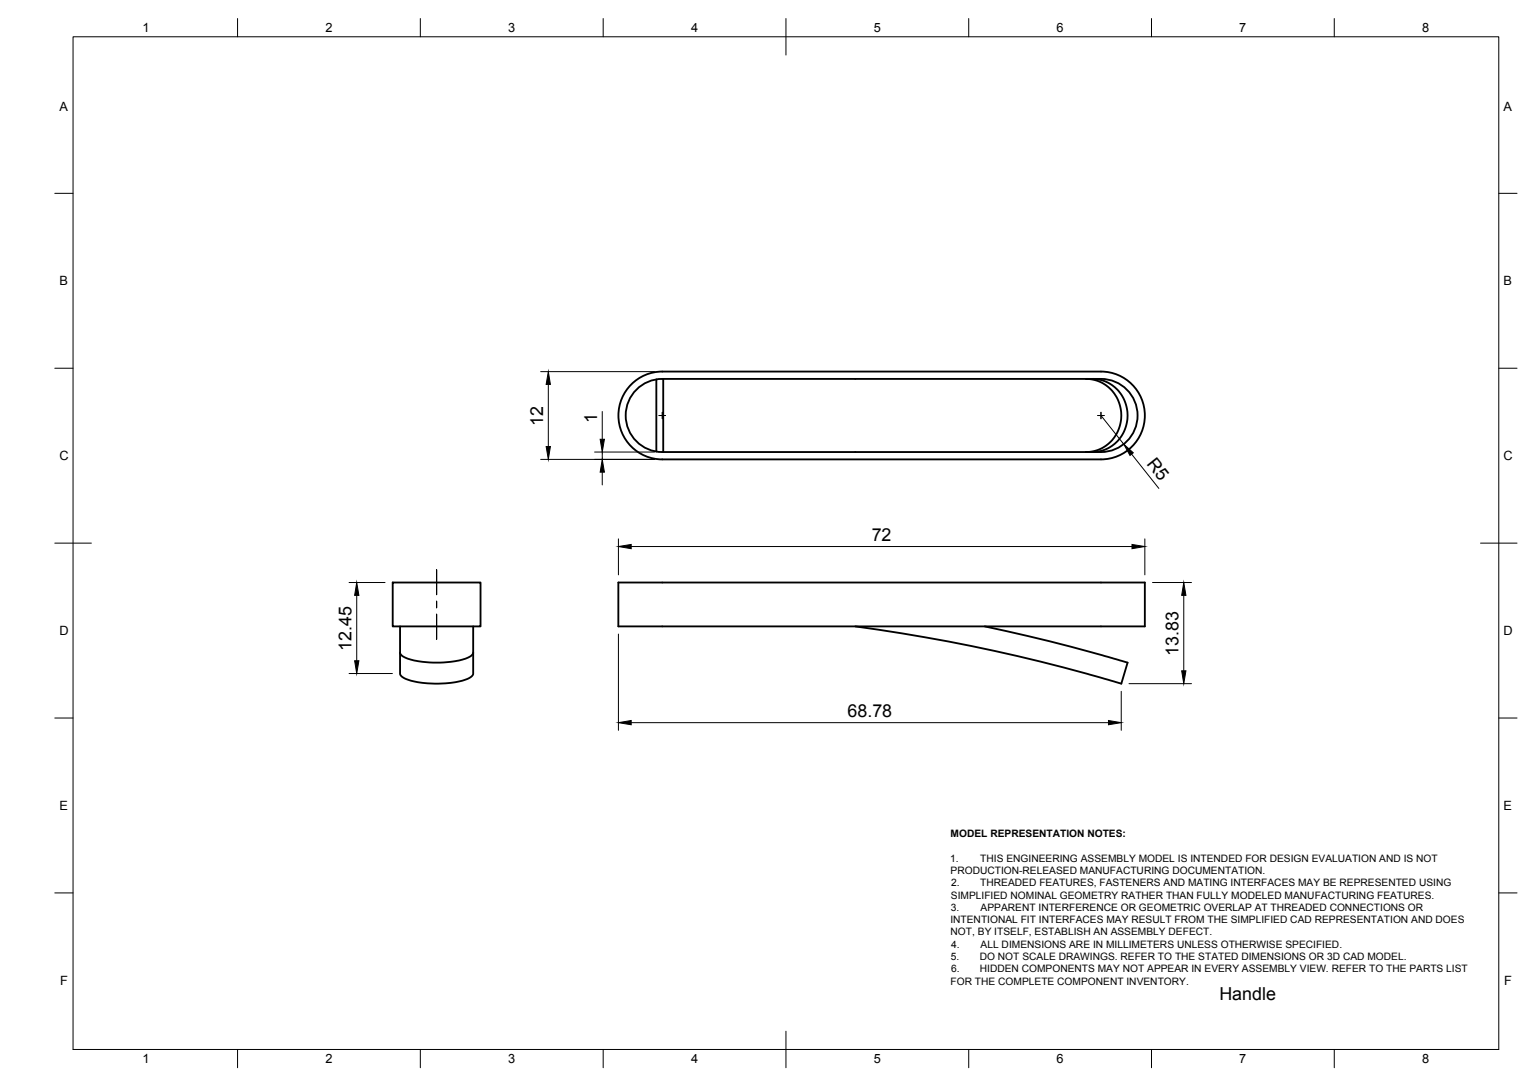
ISO-10303-21;
HEADER;
/* Generated by software containing ST-Developer
 * from STEP Tools, Inc. (www.steptools.com) 
 */

FILE_DESCRIPTION(
/* description */ (''),
/* implementation_level */ '2;1');

FILE_NAME(
/* name */ 'Handle.step',
/* time_stamp */ '2026-10-06T12:52:28-07:00',
/* author */ (''),
/* organization */ (''),
/* preprocessor_version */ 'ST-DEVELOPER v20.2',
/* originating_system */ 'Autodesk Translation Framework v15.15.0.0',
/* authorisation */ '');

FILE_SCHEMA (('AUTOMOTIVE_DESIGN { 1 0 10303 214 3 1 1 }'));
ENDSEC;

DATA;
#10=MECHANICAL_DESIGN_GEOMETRIC_PRESENTATION_REPRESENTATION('',(#80),#34403);
#43=ELLIPSE('',#4958,16.4522491302287,5.);
#44=ELLIPSE('',#4959,16.4522491302287,5.);
#64=SHAPE_REPRESENTATION_RELATIONSHIP('SRR','None',#34442,#72);
#72=ADVANCED_BREP_SHAPE_REPRESENTATION('',(#88),#34402);
#80=STYLED_ITEM('',(#34484),#88);
#88=MANIFOLD_SOLID_BREP('Body1',#4389);
#124=FACE_BOUND('',#1013,.T.);
#147=PLANE('',#4957);
#148=PLANE('',#4971);
#149=PLANE('',#4972);
#150=PLANE('',#4973);
#151=PLANE('',#4974);
#152=PLANE('',#4976);
#153=PLANE('',#4977);
#154=PLANE('',#4980);
#155=PLANE('',#4984);
#156=PLANE('',#4985);
#157=PLANE('',#4989);
#158=PLANE('',#4993);
#159=PLANE('',#4994);
#430=CIRCLE('',#4961,241.305156942645);
#431=CIRCLE('',#4962,241.305156942645);
#432=CIRCLE('',#4963,241.305156942645);
#433=CIRCLE('',#4964,241.305156942645);
#434=CIRCLE('',#4967,238.305156942645);
#435=CIRCLE('',#4968,238.305156942645);
#436=CIRCLE('',#4969,238.305156942645);
#437=CIRCLE('',#4970,238.305156942645);
#438=CIRCLE('',#4975,5.);
#439=CIRCLE('',#4979,5.);
#440=CIRCLE('',#4982,5.);
#441=CIRCLE('',#4983,5.);
#442=CIRCLE('',#4987,6.);
#443=CIRCLE('',#4988,6.);
#444=CIRCLE('',#4991,6.);
#445=CIRCLE('',#4992,6.);
#727=FACE_OUTER_BOUND('',#993,.T.);
#728=FACE_OUTER_BOUND('',#994,.T.);
#729=FACE_OUTER_BOUND('',#995,.T.);
#730=FACE_OUTER_BOUND('',#996,.T.);
#731=FACE_OUTER_BOUND('',#997,.T.);
#732=FACE_OUTER_BOUND('',#998,.T.);
#733=FACE_OUTER_BOUND('',#999,.T.);
#734=FACE_OUTER_BOUND('',#1000,.T.);
#735=FACE_OUTER_BOUND('',#1001,.T.);
#736=FACE_OUTER_BOUND('',#1002,.T.);
#737=FACE_OUTER_BOUND('',#1003,.T.);
#738=FACE_OUTER_BOUND('',#1004,.T.);
#739=FACE_OUTER_BOUND('',#1005,.T.);
#740=FACE_OUTER_BOUND('',#1006,.T.);
#741=FACE_OUTER_BOUND('',#1007,.T.);
#742=FACE_OUTER_BOUND('',#1008,.T.);
#743=FACE_OUTER_BOUND('',#1009,.T.);
#744=FACE_OUTER_BOUND('',#1010,.T.);
#745=FACE_OUTER_BOUND('',#1011,.T.);
#746=FACE_OUTER_BOUND('',#1012,.T.);
#993=EDGE_LOOP('',(#3943,#3944,#3945,#3946,#3947,#3948));
#994=EDGE_LOOP('',(#3949,#3950,#3951,#3952,#3953,#3954));
#995=EDGE_LOOP('',(#3955,#3956,#3957,#3958));
#996=EDGE_LOOP('',(#3959,#3960,#3961,#3962,#3963,#3964));
#997=EDGE_LOOP('',(#3965,#3966,#3967,#3968));
#998=EDGE_LOOP('',(#3969,#3970,#3971,#3972));
#999=EDGE_LOOP('',(#3973,#3974,#3975,#3976));
#1000=EDGE_LOOP('',(#3977,#3978,#3979,#3980));
#1001=EDGE_LOOP('',(#3981,#3982,#3983,#3984));
#1002=EDGE_LOOP('',(#3985,#3986,#3987,#3988));
#1003=EDGE_LOOP('',(#3989,#3990,#3991,#3992));
#1004=EDGE_LOOP('',(#3993,#3994,#3995,#3996));
#1005=EDGE_LOOP('',(#3997,#3998,#3999,#4000,#4001,#4002));
#1006=EDGE_LOOP('',(#4003,#4004));
#1007=EDGE_LOOP('',(#4005,#4006,#4007,#4008));
#1008=EDGE_LOOP('',(#4009,#4010,#4011,#4012));
#1009=EDGE_LOOP('',(#4013,#4014,#4015,#4016));
#1010=EDGE_LOOP('',(#4017,#4018,#4019,#4020));
#1011=EDGE_LOOP('',(#4021,#4022,#4023,#4024));
#1012=EDGE_LOOP('',(#4025,#4026,#4027,#4028));
#1013=EDGE_LOOP('',(#4029,#4030,#4031,#4032,#4033,#4034,#4035,#4036));
#1124=LINE('',#34248,#1261);
#1125=LINE('',#34252,#1262);
#1126=LINE('',#34254,#1263);
#1127=LINE('',#34255,#1264);
#1128=LINE('',#34259,#1265);
#1129=LINE('',#34309,#1266);
#1130=LINE('',#34310,#1267);
#1131=LINE('',#34319,#1268);
#1132=LINE('',#34321,#1269);
#1133=LINE('',#34324,#1270);
#1134=LINE('',#34326,#1271);
#1135=LINE('',#34327,#1272);
#1136=LINE('',#34330,#1273);
#1137=LINE('',#34334,#1274);
#1138=LINE('',#34335,#1275);
#1139=LINE('',#34338,#1276);
#1140=LINE('',#34339,#1277);
#1141=LINE('',#34344,#1278);
#1142=LINE('',#34345,#1279);
#1143=LINE('',#34353,#1280);
#1144=LINE('',#34355,#1281);
#1145=LINE('',#34357,#1282);
#1146=LINE('',#34358,#1283);
#1147=LINE('',#34364,#1284);
#1148=LINE('',#34367,#1285);
#1149=LINE('',#34369,#1286);
#1150=LINE('',#34370,#1287);
#1261=VECTOR('',#6073,10.);
#1262=VECTOR('',#6076,10.);
#1263=VECTOR('',#6077,10.);
#1264=VECTOR('',#6078,10.);
#1265=VECTOR('',#6081,10.);
#1266=VECTOR('',#6092,10.);
#1267=VECTOR('',#6093,10.);
#1268=VECTOR('',#6106,10.);
#1269=VECTOR('',#6109,10.);
#1270=VECTOR('',#6112,10.);
#1271=VECTOR('',#6113,10.);
#1272=VECTOR('',#6114,10.);
#1273=VECTOR('',#6117,10.);
#1274=VECTOR('',#6122,10.);
#1275=VECTOR('',#6123,10.);
#1276=VECTOR('',#6126,10.);
#1277=VECTOR('',#6127,10.);
#1278=VECTOR('',#6134,10.);
#1279=VECTOR('',#6135,10.);
#1280=VECTOR('',#6146,10.);
#1281=VECTOR('',#6147,10.);
#1282=VECTOR('',#6148,10.);
#1283=VECTOR('',#6149,10.);
#1284=VECTOR('',#6156,10.);
#1285=VECTOR('',#6159,10.);
#1286=VECTOR('',#6160,10.);
#1287=VECTOR('',#6161,10.);
#1538=B_SPLINE_CURVE_WITH_KNOTS('',3,(#34265,#34266,#34267,#34268,#34269,
#34270,#34271,#34272,#34273,#34274,#34275,#34276,#34277,#34278,#34279,#34280,
#34281,#34282,#34283),.UNSPECIFIED.,.F.,.F.,(4,2,2,2,3,2,2,2,4),(2.26050146390194,
2.44886175450614,2.63722204511035,2.82556593417816,3.01390982324597,3.20225371231378,
3.39059760138159,3.5789578919858,3.76731818259),.UNSPECIFIED.);
#1539=B_SPLINE_CURVE_WITH_KNOTS('',3,(#34290,#34291,#34292,#34293,#34294,
#34295,#34296,#34297,#34298,#34299,#34300,#34301,#34302,#34303,#34304,#34305,
#34306,#34307,#34308),.UNSPECIFIED.,.F.,.F.,(4,2,2,2,3,2,2,2,4),(2.26051113353486,
2.44887185347984,2.63723257342483,2.82557647618218,3.01392037893953,3.20226428169689,
3.39060818445424,3.57896890439922,3.76732962434421),.UNSPECIFIED.);
#1976=VERTEX_POINT('',#34244);
#1977=VERTEX_POINT('',#34245);
#1978=VERTEX_POINT('',#34247);
#1979=VERTEX_POINT('',#34249);
#1980=VERTEX_POINT('',#34251);
#1981=VERTEX_POINT('',#34253);
#1982=VERTEX_POINT('',#34257);
#1983=VERTEX_POINT('',#34258);
#1984=VERTEX_POINT('',#34260);
#1985=VERTEX_POINT('',#34262);
#1986=VERTEX_POINT('',#34264);
#1987=VERTEX_POINT('',#34284);
#1988=VERTEX_POINT('',#34288);
#1989=VERTEX_POINT('',#34289);
#1990=VERTEX_POINT('',#34312);
#1991=VERTEX_POINT('',#34315);
#1992=VERTEX_POINT('',#34323);
#1993=VERTEX_POINT('',#34325);
#1994=VERTEX_POINT('',#34329);
#1995=VERTEX_POINT('',#34333);
#1996=VERTEX_POINT('',#34337);
#1997=VERTEX_POINT('',#34343);
#1998=VERTEX_POINT('',#34351);
#1999=VERTEX_POINT('',#34352);
#2000=VERTEX_POINT('',#34354);
#2001=VERTEX_POINT('',#34356);
#2002=VERTEX_POINT('',#34360);
#2003=VERTEX_POINT('',#34362);
#2004=VERTEX_POINT('',#34366);
#2005=VERTEX_POINT('',#34368);
#2636=EDGE_CURVE('',#1976,#1977,#43,.T.);
#2637=EDGE_CURVE('',#1978,#1976,#1124,.T.);
#2638=EDGE_CURVE('',#1979,#1978,#44,.T.);
#2639=EDGE_CURVE('',#1980,#1979,#1125,.T.);
#2640=EDGE_CURVE('',#1980,#1981,#1126,.T.);
#2641=EDGE_CURVE('',#1977,#1981,#1127,.T.);
#2642=EDGE_CURVE('',#1982,#1983,#1128,.T.);
#2643=EDGE_CURVE('',#1984,#1982,#430,.T.);
#2644=EDGE_CURVE('',#1985,#1984,#431,.T.);
#2645=EDGE_CURVE('',#1986,#1985,#1538,.F.);
#2646=EDGE_CURVE('',#1987,#1986,#432,.T.);
#2647=EDGE_CURVE('',#1983,#1987,#433,.T.);
#2648=EDGE_CURVE('',#1988,#1989,#1539,.F.);
#2649=EDGE_CURVE('',#1989,#1986,#1129,.T.);
#2650=EDGE_CURVE('',#1985,#1988,#1130,.T.);
#2651=EDGE_CURVE('',#1990,#1988,#434,.T.);
#2652=EDGE_CURVE('',#1981,#1990,#435,.T.);
#2653=EDGE_CURVE('',#1991,#1980,#436,.T.);
#2654=EDGE_CURVE('',#1989,#1991,#437,.T.);
#2655=EDGE_CURVE('',#1987,#1991,#1131,.T.);
#2656=EDGE_CURVE('',#1990,#1984,#1132,.T.);
#2657=EDGE_CURVE('',#1982,#1992,#1133,.F.);
#2658=EDGE_CURVE('',#1993,#1992,#1134,.T.);
#2659=EDGE_CURVE('',#1984,#1993,#1135,.T.);
#2660=EDGE_CURVE('',#1994,#1983,#1136,.F.);
#2661=EDGE_CURVE('',#1992,#1994,#438,.F.);
#2662=EDGE_CURVE('',#1995,#1979,#1137,.T.);
#2663=EDGE_CURVE('',#1991,#1995,#1138,.T.);
#2664=EDGE_CURVE('',#1996,#1987,#1139,.T.);
#2665=EDGE_CURVE('',#1996,#1994,#1140,.T.);
#2666=EDGE_CURVE('',#1993,#1996,#439,.T.);
#2667=EDGE_CURVE('',#1997,#1990,#1141,.T.);
#2668=EDGE_CURVE('',#1997,#1977,#1142,.T.);
#2669=EDGE_CURVE('',#1995,#1997,#440,.T.);
#2670=EDGE_CURVE('',#1978,#1976,#441,.F.);
#2671=EDGE_CURVE('',#1998,#1999,#1143,.T.);
#2672=EDGE_CURVE('',#1999,#2000,#1144,.T.);
#2673=EDGE_CURVE('',#2001,#2000,#1145,.T.);
#2674=EDGE_CURVE('',#1998,#2001,#1146,.T.);
#2675=EDGE_CURVE('',#2002,#1998,#442,.T.);
#2676=EDGE_CURVE('',#2003,#2001,#443,.T.);
#2677=EDGE_CURVE('',#2002,#2003,#1147,.T.);
#2678=EDGE_CURVE('',#2004,#2002,#1148,.T.);
#2679=EDGE_CURVE('',#2005,#2003,#1149,.T.);
#2680=EDGE_CURVE('',#2004,#2005,#1150,.T.);
#2681=EDGE_CURVE('',#1999,#2004,#444,.T.);
#2682=EDGE_CURVE('',#2000,#2005,#445,.T.);
#3943=ORIENTED_EDGE('',*,*,#2636,.F.);
#3944=ORIENTED_EDGE('',*,*,#2637,.F.);
#3945=ORIENTED_EDGE('',*,*,#2638,.F.);
#3946=ORIENTED_EDGE('',*,*,#2639,.F.);
#3947=ORIENTED_EDGE('',*,*,#2640,.T.);
#3948=ORIENTED_EDGE('',*,*,#2641,.F.);
#3949=ORIENTED_EDGE('',*,*,#2642,.F.);
#3950=ORIENTED_EDGE('',*,*,#2643,.F.);
#3951=ORIENTED_EDGE('',*,*,#2644,.F.);
#3952=ORIENTED_EDGE('',*,*,#2645,.F.);
#3953=ORIENTED_EDGE('',*,*,#2646,.F.);
#3954=ORIENTED_EDGE('',*,*,#2647,.F.);
#3955=ORIENTED_EDGE('',*,*,#2648,.T.);
#3956=ORIENTED_EDGE('',*,*,#2649,.T.);
#3957=ORIENTED_EDGE('',*,*,#2645,.T.);
#3958=ORIENTED_EDGE('',*,*,#2650,.T.);
#3959=ORIENTED_EDGE('',*,*,#2648,.F.);
#3960=ORIENTED_EDGE('',*,*,#2651,.F.);
#3961=ORIENTED_EDGE('',*,*,#2652,.F.);
#3962=ORIENTED_EDGE('',*,*,#2640,.F.);
#3963=ORIENTED_EDGE('',*,*,#2653,.F.);
#3964=ORIENTED_EDGE('',*,*,#2654,.F.);
#3965=ORIENTED_EDGE('',*,*,#2655,.F.);
#3966=ORIENTED_EDGE('',*,*,#2646,.T.);
#3967=ORIENTED_EDGE('',*,*,#2649,.F.);
#3968=ORIENTED_EDGE('',*,*,#2654,.T.);
#3969=ORIENTED_EDGE('',*,*,#2656,.F.);
#3970=ORIENTED_EDGE('',*,*,#2651,.T.);
#3971=ORIENTED_EDGE('',*,*,#2650,.F.);
#3972=ORIENTED_EDGE('',*,*,#2644,.T.);
#3973=ORIENTED_EDGE('',*,*,#2643,.T.);
#3974=ORIENTED_EDGE('',*,*,#2657,.T.);
#3975=ORIENTED_EDGE('',*,*,#2658,.F.);
#3976=ORIENTED_EDGE('',*,*,#2659,.F.);
#3977=ORIENTED_EDGE('',*,*,#2642,.T.);
#3978=ORIENTED_EDGE('',*,*,#2660,.F.);
#3979=ORIENTED_EDGE('',*,*,#2661,.F.);
#3980=ORIENTED_EDGE('',*,*,#2657,.F.);
#3981=ORIENTED_EDGE('',*,*,#2653,.T.);
#3982=ORIENTED_EDGE('',*,*,#2639,.T.);
#3983=ORIENTED_EDGE('',*,*,#2662,.F.);
#3984=ORIENTED_EDGE('',*,*,#2663,.F.);
#3985=ORIENTED_EDGE('',*,*,#2647,.T.);
#3986=ORIENTED_EDGE('',*,*,#2664,.F.);
#3987=ORIENTED_EDGE('',*,*,#2665,.T.);
#3988=ORIENTED_EDGE('',*,*,#2660,.T.);
#3989=ORIENTED_EDGE('',*,*,#2666,.F.);
#3990=ORIENTED_EDGE('',*,*,#2658,.T.);
#3991=ORIENTED_EDGE('',*,*,#2661,.T.);
#3992=ORIENTED_EDGE('',*,*,#2665,.F.);
#3993=ORIENTED_EDGE('',*,*,#2652,.T.);
#3994=ORIENTED_EDGE('',*,*,#2667,.F.);
#3995=ORIENTED_EDGE('',*,*,#2668,.T.);
#3996=ORIENTED_EDGE('',*,*,#2641,.T.);
#3997=ORIENTED_EDGE('',*,*,#2636,.T.);
#3998=ORIENTED_EDGE('',*,*,#2668,.F.);
#3999=ORIENTED_EDGE('',*,*,#2669,.F.);
#4000=ORIENTED_EDGE('',*,*,#2662,.T.);
#4001=ORIENTED_EDGE('',*,*,#2638,.T.);
#4002=ORIENTED_EDGE('',*,*,#2670,.T.);
#4003=ORIENTED_EDGE('',*,*,#2637,.T.);
#4004=ORIENTED_EDGE('',*,*,#2670,.F.);
#4005=ORIENTED_EDGE('',*,*,#2671,.T.);
#4006=ORIENTED_EDGE('',*,*,#2672,.T.);
#4007=ORIENTED_EDGE('',*,*,#2673,.F.);
#4008=ORIENTED_EDGE('',*,*,#2674,.F.);
#4009=ORIENTED_EDGE('',*,*,#2675,.T.);
#4010=ORIENTED_EDGE('',*,*,#2674,.T.);
#4011=ORIENTED_EDGE('',*,*,#2676,.F.);
#4012=ORIENTED_EDGE('',*,*,#2677,.F.);
#4013=ORIENTED_EDGE('',*,*,#2678,.T.);
#4014=ORIENTED_EDGE('',*,*,#2677,.T.);
#4015=ORIENTED_EDGE('',*,*,#2679,.F.);
#4016=ORIENTED_EDGE('',*,*,#2680,.F.);
#4017=ORIENTED_EDGE('',*,*,#2681,.T.);
#4018=ORIENTED_EDGE('',*,*,#2680,.T.);
#4019=ORIENTED_EDGE('',*,*,#2682,.F.);
#4020=ORIENTED_EDGE('',*,*,#2672,.F.);
#4021=ORIENTED_EDGE('',*,*,#2682,.T.);
#4022=ORIENTED_EDGE('',*,*,#2679,.T.);
#4023=ORIENTED_EDGE('',*,*,#2676,.T.);
#4024=ORIENTED_EDGE('',*,*,#2673,.T.);
#4025=ORIENTED_EDGE('',*,*,#2681,.F.);
#4026=ORIENTED_EDGE('',*,*,#2671,.F.);
#4027=ORIENTED_EDGE('',*,*,#2675,.F.);
#4028=ORIENTED_EDGE('',*,*,#2678,.F.);
#4029=ORIENTED_EDGE('',*,*,#2664,.T.);
#4030=ORIENTED_EDGE('',*,*,#2655,.T.);
#4031=ORIENTED_EDGE('',*,*,#2663,.T.);
#4032=ORIENTED_EDGE('',*,*,#2669,.T.);
#4033=ORIENTED_EDGE('',*,*,#2667,.T.);
#4034=ORIENTED_EDGE('',*,*,#2656,.T.);
#4035=ORIENTED_EDGE('',*,*,#2659,.T.);
#4036=ORIENTED_EDGE('',*,*,#2666,.T.);
#4144=CYLINDRICAL_SURFACE('',#4960,241.305156942645);
#4145=CYLINDRICAL_SURFACE('',#4965,5.);
#4146=CYLINDRICAL_SURFACE('',#4966,238.305156942645);
#4147=CYLINDRICAL_SURFACE('',#4978,5.);
#4148=CYLINDRICAL_SURFACE('',#4981,5.);
#4149=CYLINDRICAL_SURFACE('',#4986,6.);
#4150=CYLINDRICAL_SURFACE('',#4990,6.);
#4362=ADVANCED_FACE('',(#727),#147,.T.);
#4363=ADVANCED_FACE('',(#728),#4144,.T.);
#4364=ADVANCED_FACE('',(#729),#4145,.T.);
#4365=ADVANCED_FACE('',(#730),#4146,.F.);
#4366=ADVANCED_FACE('',(#731),#148,.F.);
#4367=ADVANCED_FACE('',(#732),#149,.T.);
#4368=ADVANCED_FACE('',(#733),#150,.F.);
#4369=ADVANCED_FACE('',(#734),#151,.F.);
#4370=ADVANCED_FACE('',(#735),#152,.F.);
#4371=ADVANCED_FACE('',(#736),#153,.F.);
#4372=ADVANCED_FACE('',(#737),#4147,.F.);
#4373=ADVANCED_FACE('',(#738),#154,.F.);
#4374=ADVANCED_FACE('',(#739),#4148,.F.);
#4375=ADVANCED_FACE('',(#740),#155,.F.);
#4376=ADVANCED_FACE('',(#741),#156,.T.);
#4377=ADVANCED_FACE('',(#742),#4149,.T.);
#4378=ADVANCED_FACE('',(#743),#157,.T.);
#4379=ADVANCED_FACE('',(#744),#4150,.T.);
#4380=ADVANCED_FACE('',(#745),#158,.T.);
#4381=ADVANCED_FACE('',(#746,#124),#159,.F.);
#4389=CLOSED_SHELL('',(#4362,#4363,#4364,#4365,#4366,#4367,#4368,#4369,
#4370,#4371,#4372,#4373,#4374,#4375,#4376,#4377,#4378,#4379,#4380,#4381));
#4956=AXIS2_PLACEMENT_3D('',#34242,#6067,#6068);
#4957=AXIS2_PLACEMENT_3D('',#34243,#6069,#6070);
#4958=AXIS2_PLACEMENT_3D('',#34246,#6071,#6072);
#4959=AXIS2_PLACEMENT_3D('',#34250,#6074,#6075);
#4960=AXIS2_PLACEMENT_3D('',#34256,#6079,#6080);
#4961=AXIS2_PLACEMENT_3D('',#34261,#6082,#6083);
#4962=AXIS2_PLACEMENT_3D('',#34263,#6084,#6085);
#4963=AXIS2_PLACEMENT_3D('',#34285,#6086,#6087);
#4964=AXIS2_PLACEMENT_3D('',#34286,#6088,#6089);
#4965=AXIS2_PLACEMENT_3D('',#34287,#6090,#6091);
#4966=AXIS2_PLACEMENT_3D('',#34311,#6094,#6095);
#4967=AXIS2_PLACEMENT_3D('',#34313,#6096,#6097);
#4968=AXIS2_PLACEMENT_3D('',#34314,#6098,#6099);
#4969=AXIS2_PLACEMENT_3D('',#34316,#6100,#6101);
#4970=AXIS2_PLACEMENT_3D('',#34317,#6102,#6103);
#4971=AXIS2_PLACEMENT_3D('',#34318,#6104,#6105);
#4972=AXIS2_PLACEMENT_3D('',#34320,#6107,#6108);
#4973=AXIS2_PLACEMENT_3D('',#34322,#6110,#6111);
#4974=AXIS2_PLACEMENT_3D('',#34328,#6115,#6116);
#4975=AXIS2_PLACEMENT_3D('',#34331,#6118,#6119);
#4976=AXIS2_PLACEMENT_3D('',#34332,#6120,#6121);
#4977=AXIS2_PLACEMENT_3D('',#34336,#6124,#6125);
#4978=AXIS2_PLACEMENT_3D('',#34340,#6128,#6129);
#4979=AXIS2_PLACEMENT_3D('',#34341,#6130,#6131);
#4980=AXIS2_PLACEMENT_3D('',#34342,#6132,#6133);
#4981=AXIS2_PLACEMENT_3D('',#34346,#6136,#6137);
#4982=AXIS2_PLACEMENT_3D('',#34347,#6138,#6139);
#4983=AXIS2_PLACEMENT_3D('',#34348,#6140,#6141);
#4984=AXIS2_PLACEMENT_3D('',#34349,#6142,#6143);
#4985=AXIS2_PLACEMENT_3D('',#34350,#6144,#6145);
#4986=AXIS2_PLACEMENT_3D('',#34359,#6150,#6151);
#4987=AXIS2_PLACEMENT_3D('',#34361,#6152,#6153);
#4988=AXIS2_PLACEMENT_3D('',#34363,#6154,#6155);
#4989=AXIS2_PLACEMENT_3D('',#34365,#6157,#6158);
#4990=AXIS2_PLACEMENT_3D('',#34371,#6162,#6163);
#4991=AXIS2_PLACEMENT_3D('',#34372,#6164,#6165);
#4992=AXIS2_PLACEMENT_3D('',#34373,#6166,#6167);
#4993=AXIS2_PLACEMENT_3D('',#34374,#6168,#6169);
#4994=AXIS2_PLACEMENT_3D('',#34375,#6170,#6171);
#6067=DIRECTION('axis',(0.,0.,1.));
#6068=DIRECTION('refdir',(1.,0.,0.));
#6069=DIRECTION('center_axis',(0.952700805058341,0.,-0.303909815638107));
#6070=DIRECTION('ref_axis',(-0.303909815638107,0.,-0.952700805058341));
#6071=DIRECTION('center_axis',(-0.952700805058341,0.,0.303909815638107));
#6072=DIRECTION('ref_axis',(0.303909815638107,0.,0.952700805058341));
#6073=DIRECTION('',(0.,1.,0.));
#6074=DIRECTION('center_axis',(-0.952700805058341,0.,0.303909815638107));
#6075=DIRECTION('ref_axis',(0.303909815638107,0.,0.952700805058341));
#6076=DIRECTION('',(0.303909815638107,0.,0.952700805058341));
#6077=DIRECTION('',(0.,1.,0.));
#6078=DIRECTION('',(-0.303909815638107,0.,-0.952700805058341));
#6079=DIRECTION('center_axis',(0.,1.,0.));
#6080=DIRECTION('ref_axis',(-0.286009483054508,0.,0.958226787145346));
#6081=DIRECTION('',(0.,-1.,0.));
#6082=DIRECTION('center_axis',(0.,1.,0.));
#6083=DIRECTION('ref_axis',(-0.286009483054508,0.,0.958226787145346));
#6084=DIRECTION('center_axis',(0.,1.,0.));
#6085=DIRECTION('ref_axis',(-0.286009483054508,0.,0.958226787145346));
#6086=DIRECTION('center_axis',(0.,-1.,0.));
#6087=DIRECTION('ref_axis',(-0.286009483054508,0.,0.958226787145346));
#6088=DIRECTION('center_axis',(0.,-1.,0.));
#6089=DIRECTION('ref_axis',(-0.286009483054508,0.,0.958226787145346));
#6090=DIRECTION('center_axis',(0.286009483054514,0.,-0.958226787145345));
#6091=DIRECTION('ref_axis',(-0.677568659105072,-0.707106781186547,-0.202239244951506));
#6092=DIRECTION('',(-0.286009483054514,0.,0.958226787145345));
#6093=DIRECTION('',(0.286009483054514,0.,-0.958226787145345));
#6094=DIRECTION('center_axis',(0.,1.,0.));
#6095=DIRECTION('ref_axis',(-0.286009483054508,0.,0.958226787145346));
#6096=DIRECTION('center_axis',(0.,-1.,0.));
#6097=DIRECTION('ref_axis',(-0.286009483054508,0.,0.958226787145346));
#6098=DIRECTION('center_axis',(0.,-1.,0.));
#6099=DIRECTION('ref_axis',(-0.286009483054508,0.,0.958226787145346));
#6100=DIRECTION('center_axis',(0.,1.,0.));
#6101=DIRECTION('ref_axis',(-0.286009483054508,0.,0.958226787145346));
#6102=DIRECTION('center_axis',(0.,1.,0.));
#6103=DIRECTION('ref_axis',(-0.286009483054508,0.,0.958226787145346));
#6104=DIRECTION('center_axis',(0.,1.,0.));
#6105=DIRECTION('ref_axis',(1.,0.,0.));
#6106=DIRECTION('',(1.,0.,0.));
#6107=DIRECTION('center_axis',(0.,1.,0.));
#6108=DIRECTION('ref_axis',(1.,0.,0.));
#6109=DIRECTION('',(-1.,0.,0.));
#6110=DIRECTION('center_axis',(0.,1.,0.));
#6111=DIRECTION('ref_axis',(-1.,0.,0.));
#6112=DIRECTION('',(1.,0.,0.));
#6113=DIRECTION('',(0.,0.,1.));
#6114=DIRECTION('',(-1.,0.,0.));
#6115=DIRECTION('center_axis',(0.,0.,1.));
#6116=DIRECTION('ref_axis',(-1.,0.,0.));
#6117=DIRECTION('',(-1.,0.,0.));
#6118=DIRECTION('center_axis',(0.,0.,-1.));
#6119=DIRECTION('ref_axis',(0.,1.,0.));
#6120=DIRECTION('center_axis',(0.,-1.,0.));
#6121=DIRECTION('ref_axis',(1.,0.,0.));
#6122=DIRECTION('',(0.,0.,1.));
#6123=DIRECTION('',(1.,0.,0.));
#6124=DIRECTION('center_axis',(0.,-1.,0.));
#6125=DIRECTION('ref_axis',(1.,0.,0.));
#6126=DIRECTION('',(1.,0.,0.));
#6127=DIRECTION('',(0.,0.,1.));
#6128=DIRECTION('center_axis',(0.,0.,1.));
#6129=DIRECTION('ref_axis',(0.,1.,0.));
#6130=DIRECTION('center_axis',(0.,0.,1.));
#6131=DIRECTION('ref_axis',(0.,1.,0.));
#6132=DIRECTION('center_axis',(0.,1.,0.));
#6133=DIRECTION('ref_axis',(-1.,0.,0.));
#6134=DIRECTION('',(-1.,0.,0.));
#6135=DIRECTION('',(0.,0.,1.));
#6136=DIRECTION('center_axis',(0.,0.,1.));
#6137=DIRECTION('ref_axis',(0.,-1.,0.));
#6138=DIRECTION('center_axis',(0.,0.,1.));
#6139=DIRECTION('ref_axis',(0.,-1.,0.));
#6140=DIRECTION('center_axis',(0.,0.,-1.));
#6141=DIRECTION('ref_axis',(0.,-1.,0.));
#6142=DIRECTION('center_axis',(0.,0.,1.));
#6143=DIRECTION('ref_axis',(-1.,0.,0.));
#6144=DIRECTION('center_axis',(0.,-1.,0.));
#6145=DIRECTION('ref_axis',(1.,0.,0.));
#6146=DIRECTION('',(1.,0.,0.));
#6147=DIRECTION('',(0.,0.,1.));
#6148=DIRECTION('',(1.,0.,0.));
#6149=DIRECTION('',(0.,0.,1.));
#6150=DIRECTION('center_axis',(0.,0.,1.));
#6151=DIRECTION('ref_axis',(0.,1.,0.));
#6152=DIRECTION('center_axis',(0.,0.,1.));
#6153=DIRECTION('ref_axis',(0.,1.,0.));
#6154=DIRECTION('center_axis',(0.,0.,1.));
#6155=DIRECTION('ref_axis',(0.,1.,0.));
#6156=DIRECTION('',(0.,0.,1.));
#6157=DIRECTION('center_axis',(0.,1.,0.));
#6158=DIRECTION('ref_axis',(-1.,0.,0.));
#6159=DIRECTION('',(-1.,0.,0.));
#6160=DIRECTION('',(-1.,0.,0.));
#6161=DIRECTION('',(0.,0.,1.));
#6162=DIRECTION('center_axis',(0.,0.,1.));
#6163=DIRECTION('ref_axis',(0.,-1.,0.));
#6164=DIRECTION('center_axis',(0.,0.,1.));
#6165=DIRECTION('ref_axis',(0.,-1.,0.));
#6166=DIRECTION('center_axis',(0.,0.,1.));
#6167=DIRECTION('ref_axis',(0.,-1.,0.));
#6168=DIRECTION('center_axis',(0.,0.,1.));
#6169=DIRECTION('ref_axis',(-1.,0.,0.));
#6170=DIRECTION('center_axis',(0.,0.,1.));
#6171=DIRECTION('ref_axis',(-1.,0.,0.));
#34242=CARTESIAN_POINT('',(0.,0.,0.));
#34243=CARTESIAN_POINT('Origin',(0.830812522453709,0.,65.2859978089105));
#34244=CARTESIAN_POINT('',(0.803379378582617,4.93503612692635,65.2));
#34245=CARTESIAN_POINT('',(7.34788079488412E-16,5.,62.6815549174156));
#34246=CARTESIAN_POINT('Origin',(0.,0.,62.6815549174156));
#34247=CARTESIAN_POINT('',(0.803379378582617,-4.93503612692635,65.2));
#34248=CARTESIAN_POINT('',(0.803379378582612,0.,65.2));
#34249=CARTESIAN_POINT('',(0.,-5.,62.6815549174156));
#34250=CARTESIAN_POINT('Origin',(0.,0.,62.6815549174156));
#34251=CARTESIAN_POINT('',(-0.132842333122278,-5.,62.2651188854115));
#34252=CARTESIAN_POINT('',(-2.71467767788293,-5.,54.1715447890402));
#34253=CARTESIAN_POINT('',(-0.132842333122278,5.,62.2651188854115));
#34254=CARTESIAN_POINT('',(-0.132842333122279,0.,62.2651188854115));
#34255=CARTESIAN_POINT('',(0.0561576033527066,5.,62.8575985697469));
#34256=CARTESIAN_POINT('Origin',(5.37767154318555,0.,-175.976317607651));
#34257=CARTESIAN_POINT('',(-2.50665419388694,5.,65.2));
#34258=CARTESIAN_POINT('',(-2.50665419388694,-5.,65.2));
#34259=CARTESIAN_POINT('',(-2.50665419388694,0.,65.2));
#34260=CARTESIAN_POINT('',(-44.1089505723395,5.,60.2));
#34261=CARTESIAN_POINT('Origin',(5.37767154318555,5.,-175.976317607651));
#34262=CARTESIAN_POINT('',(-58.8319403691538,5.,56.6291520296333));
#34263=CARTESIAN_POINT('Origin',(5.37767154318555,5.,-175.976317607651));
#34264=CARTESIAN_POINT('',(-58.8319403691538,-5.,56.6291520296333));
#34265=CARTESIAN_POINT('Ctrl Pts',(-58.8319403691537,5.,56.6291520296327));
#34266=CARTESIAN_POINT('Ctrl Pts',(-59.4371717203624,5.,56.462080850099));
#34267=CARTESIAN_POINT('Ctrl Pts',(-60.0820298794635,4.8745596841293,56.2812672524265));
#34268=CARTESIAN_POINT('Ctrl Pts',(-61.2669951292512,4.36431020272779,55.9440278549618));
#34269=CARTESIAN_POINT('Ctrl Pts',(-61.8071398573752,3.97949928040823,55.787736975236));
#34270=CARTESIAN_POINT('Ctrl Pts',(-62.6594830508905,3.09160718989329,55.538954977214));
#34271=CARTESIAN_POINT('Ctrl Pts',(-63.0285088739547,2.52936940640579,55.4299017162816));
#34272=CARTESIAN_POINT('Ctrl Pts',(-63.5176931208654,1.2974722333072,55.2847309692003));
#34273=CARTESIAN_POINT('Ctrl Pts',(-63.6378916523671,0.627812963559375,
55.2487476511034));
#34274=CARTESIAN_POINT('Ctrl Pts',(-63.6378916523671,0.,55.2487476511034));
#34275=CARTESIAN_POINT('Ctrl Pts',(-63.6378916523671,-0.627812963559374,
55.2487476511034));
#34276=CARTESIAN_POINT('Ctrl Pts',(-63.5176931208654,-1.29747223330721,
55.2847309692003));
#34277=CARTESIAN_POINT('Ctrl Pts',(-63.0285088739547,-2.52936940640579,
55.4299017162816));
#34278=CARTESIAN_POINT('Ctrl Pts',(-62.6594830508905,-3.09160718989328,
55.538954977214));
#34279=CARTESIAN_POINT('Ctrl Pts',(-61.8071398573752,-3.97949928040822,
55.787736975236));
#34280=CARTESIAN_POINT('Ctrl Pts',(-61.2669951292511,-4.36431020272779,
55.9440278549618));
#34281=CARTESIAN_POINT('Ctrl Pts',(-60.0820298794635,-4.8745596841293,56.2812672524264));
#34282=CARTESIAN_POINT('Ctrl Pts',(-59.4371717203624,-5.,56.462080850099));
#34283=CARTESIAN_POINT('Ctrl Pts',(-58.8319403691537,-5.,56.6291520296327));
#34284=CARTESIAN_POINT('',(-44.1089505723395,-5.,60.2));
#34285=CARTESIAN_POINT('Origin',(5.37767154318555,-5.,-175.976317607651));
#34286=CARTESIAN_POINT('Origin',(5.37767154318555,-5.,-175.976317607651));
#34287=CARTESIAN_POINT('Origin',(-57.5900824922669,0.,52.468515568381));
#34288=CARTESIAN_POINT('',(-57.973725345055,5.,53.7538465801794));
#34289=CARTESIAN_POINT('',(-57.973725345055,-5.,53.7538465801794));
#34290=CARTESIAN_POINT('Ctrl Pts',(-57.9737253450549,-5.,53.753846580179));
#34291=CARTESIAN_POINT('Ctrl Pts',(-58.5790016453339,-5.,53.5869329349396));
#34292=CARTESIAN_POINT('Ctrl Pts',(-59.2238994944327,-4.8745603906429,53.4062543439228));
#34293=CARTESIAN_POINT('Ctrl Pts',(-60.408922048283,-4.36431138570487,53.0692049403301));
#34294=CARTESIAN_POINT('Ctrl Pts',(-60.9490848335127,-3.97950018878322,
52.9129707557609));
#34295=CARTESIAN_POINT('Ctrl Pts',(-61.8014482334478,-3.09160726119939,
52.6642535292407));
#34296=CARTESIAN_POINT('Ctrl Pts',(-62.1704778415824,-2.52936950626686,
52.5552128954911));
#34297=CARTESIAN_POINT('Ctrl Pts',(-62.6596650198333,-1.2974723188127,52.4100518473254));
#34298=CARTESIAN_POINT('Ctrl Pts',(-62.7798632032036,-0.627813009191178,
52.3740672896673));
#34299=CARTESIAN_POINT('Ctrl Pts',(-62.7798632032036,0.,52.3740672896673));
#34300=CARTESIAN_POINT('Ctrl Pts',(-62.7798632032036,0.627813009191178,
52.3740672896673));
#34301=CARTESIAN_POINT('Ctrl Pts',(-62.6596650198333,1.2974723188127,52.4100518473254));
#34302=CARTESIAN_POINT('Ctrl Pts',(-62.1704778415824,2.52936950626686,52.5552128954911));
#34303=CARTESIAN_POINT('Ctrl Pts',(-61.8014482334478,3.09160726119939,52.6642535292407));
#34304=CARTESIAN_POINT('Ctrl Pts',(-60.9490848335127,3.97950018878322,52.9129707557609));
#34305=CARTESIAN_POINT('Ctrl Pts',(-60.4089220482829,4.36431138570488,53.0692049403301));
#34306=CARTESIAN_POINT('Ctrl Pts',(-59.2238994944327,4.8745603906429,53.4062543439228));
#34307=CARTESIAN_POINT('Ctrl Pts',(-58.5790016453339,5.,53.5869329349396));
#34308=CARTESIAN_POINT('Ctrl Pts',(-57.9737253450549,5.,53.753846580179));
#34309=CARTESIAN_POINT('',(-57.5900824922669,-5.,52.468515568381));
#34310=CARTESIAN_POINT('',(-57.5900824922669,5.,52.468515568381));
#34311=CARTESIAN_POINT('Origin',(5.37767154318555,0.,-175.976317607651));
#34312=CARTESIAN_POINT('',(-26.4043174875352,5.,60.2));
#34313=CARTESIAN_POINT('Origin',(5.37767154318555,5.,-175.976317607651));
#34314=CARTESIAN_POINT('Origin',(5.37767154318555,5.,-175.976317607651));
#34315=CARTESIAN_POINT('',(-26.4043174875352,-5.,60.2));
#34316=CARTESIAN_POINT('Origin',(5.37767154318555,-5.,-175.976317607651));
#34317=CARTESIAN_POINT('Origin',(5.37767154318555,-5.,-175.976317607651));
#34318=CARTESIAN_POINT('Origin',(-31.4035395649567,-5.,58.8300325492891));
#34319=CARTESIAN_POINT('',(-45.,-5.,60.2));
#34320=CARTESIAN_POINT('Origin',(-31.4035395649567,5.,58.8300325492891));
#34321=CARTESIAN_POINT('',(-15.,5.,60.2));
#34322=CARTESIAN_POINT('Origin',(-3.67394039744206E-16,5.,60.2));
#34323=CARTESIAN_POINT('',(-60.,5.,65.2));
#34324=CARTESIAN_POINT('',(-15.,5.,65.2));
#34325=CARTESIAN_POINT('',(-60.,5.,60.2));
#34326=CARTESIAN_POINT('',(-60.,5.,60.2));
#34327=CARTESIAN_POINT('',(-15.,5.,60.2));
#34328=CARTESIAN_POINT('Origin',(-30.,0.,65.2));
#34329=CARTESIAN_POINT('',(-60.,-5.,65.2));
#34330=CARTESIAN_POINT('',(-45.,-5.,65.2));
#34331=CARTESIAN_POINT('Origin',(-60.,0.,65.2));
#34332=CARTESIAN_POINT('Origin',(-60.,-5.,60.2));
#34333=CARTESIAN_POINT('',(0.,-5.,60.2));
#34334=CARTESIAN_POINT('',(0.,-5.,60.2));
#34335=CARTESIAN_POINT('',(-45.,-5.,60.2));
#34336=CARTESIAN_POINT('Origin',(-60.,-5.,60.2));
#34337=CARTESIAN_POINT('',(-60.,-5.,60.2));
#34338=CARTESIAN_POINT('',(-45.,-5.,60.2));
#34339=CARTESIAN_POINT('',(-60.,-5.,60.2));
#34340=CARTESIAN_POINT('Origin',(-60.,0.,60.2));
#34341=CARTESIAN_POINT('Origin',(-60.,0.,60.2));
#34342=CARTESIAN_POINT('Origin',(-3.67394039744206E-16,5.,60.2));
#34343=CARTESIAN_POINT('',(3.67394039744206E-16,5.,60.2));
#34344=CARTESIAN_POINT('',(-15.,5.,60.2));
#34345=CARTESIAN_POINT('',(7.34788079488412E-16,5.,60.2));
#34346=CARTESIAN_POINT('Origin',(0.,0.,60.2));
#34347=CARTESIAN_POINT('Origin',(0.,0.,60.2));
#34348=CARTESIAN_POINT('Origin',(0.,0.,65.2));
#34349=CARTESIAN_POINT('Origin',(-30.,0.,65.2));
#34350=CARTESIAN_POINT('Origin',(-60.,-6.,60.2));
#34351=CARTESIAN_POINT('',(-60.,-6.,60.2));
#34352=CARTESIAN_POINT('',(0.,-6.,60.2));
#34353=CARTESIAN_POINT('',(-60.,-6.,60.2));
#34354=CARTESIAN_POINT('',(0.,-6.,66.2));
#34355=CARTESIAN_POINT('',(0.,-6.,60.2));
#34356=CARTESIAN_POINT('',(-60.,-6.,66.2));
#34357=CARTESIAN_POINT('',(-60.,-6.,66.2));
#34358=CARTESIAN_POINT('',(-60.,-6.,60.2));
#34359=CARTESIAN_POINT('Origin',(-60.,0.,60.2));
#34360=CARTESIAN_POINT('',(-60.,6.,60.2));
#34361=CARTESIAN_POINT('Origin',(-60.,0.,60.2));
#34362=CARTESIAN_POINT('',(-60.,6.,66.2));
#34363=CARTESIAN_POINT('Origin',(-60.,0.,66.2));
#34364=CARTESIAN_POINT('',(-60.,6.,60.2));
#34365=CARTESIAN_POINT('Origin',(-3.67394039744206E-16,6.,60.2));
#34366=CARTESIAN_POINT('',(7.34788079488412E-16,6.,60.2));
#34367=CARTESIAN_POINT('',(-3.67394039744206E-16,6.,60.2));
#34368=CARTESIAN_POINT('',(7.34788079488412E-16,6.,66.2));
#34369=CARTESIAN_POINT('',(-3.67394039744206E-16,6.,66.2));
#34370=CARTESIAN_POINT('',(7.34788079488412E-16,6.,60.2));
#34371=CARTESIAN_POINT('Origin',(0.,0.,60.2));
#34372=CARTESIAN_POINT('Origin',(0.,0.,60.2));
#34373=CARTESIAN_POINT('Origin',(0.,0.,66.2));
#34374=CARTESIAN_POINT('Origin',(-30.,0.,66.2));
#34375=CARTESIAN_POINT('Origin',(-30.,0.,60.2));
#34392=UNCERTAINTY_MEASURE_WITH_UNIT(LENGTH_MEASURE(0.01),#34404,
'DISTANCE_ACCURACY_VALUE',
'Maximum model space distance between geometric entities at asserted c
onnectivities');
#34393=UNCERTAINTY_MEASURE_WITH_UNIT(LENGTH_MEASURE(0.01),#34404,
'DISTANCE_ACCURACY_VALUE',
'Maximum model space distance between geometric entities at asserted c
onnectivities');
#34402=(
GEOMETRIC_REPRESENTATION_CONTEXT(3)
GLOBAL_UNCERTAINTY_ASSIGNED_CONTEXT((#34392))
GLOBAL_UNIT_ASSIGNED_CONTEXT((#34404,#34406,#34407))
REPRESENTATION_CONTEXT('','3D')
);
#34403=(
GEOMETRIC_REPRESENTATION_CONTEXT(3)
GLOBAL_UNCERTAINTY_ASSIGNED_CONTEXT((#34393))
GLOBAL_UNIT_ASSIGNED_CONTEXT((#34404,#34406,#34407))
REPRESENTATION_CONTEXT('','3D')
);
#34404=(
LENGTH_UNIT()
NAMED_UNIT(*)
SI_UNIT(.MILLI.,.METRE.)
);
#34406=(
NAMED_UNIT(*)
PLANE_ANGLE_UNIT()
SI_UNIT($,.RADIAN.)
);
#34407=(
NAMED_UNIT(*)
SI_UNIT($,.STERADIAN.)
SOLID_ANGLE_UNIT()
);
#34416=SHAPE_DEFINITION_REPRESENTATION(#34425,#34442);
#34425=PRODUCT_DEFINITION_SHAPE('',$,#34452);
#34442=SHAPE_REPRESENTATION('',(#4956),#34402);
#34443=PRODUCT_DEFINITION_CONTEXT('part definition',#34472,'design');
#34452=PRODUCT_DEFINITION('Handle','Handle',#34461,#34443);
#34461=PRODUCT_DEFINITION_FORMATION('',$,#34482);
#34472=APPLICATION_CONTEXT(
'Core Data for Automotive Mechanical Design Process');
#34473=PRODUCT_CONTEXT('part definition',#34472,'mechanical');
#34482=PRODUCT('Handle','Handle',$,(#34473));
#34484=PRESENTATION_STYLE_ASSIGNMENT((#34486));
#34486=SURFACE_STYLE_USAGE(.BOTH.,#34488);
#34488=SURFACE_SIDE_STYLE('',(#34490));
#34490=SURFACE_STYLE_FILL_AREA(#34492);
#34492=FILL_AREA_STYLE('Opaque(160,160,160)',(#34494));
#34494=FILL_AREA_STYLE_COLOUR('Opaque(160,160,160)',#34496);
#34496=COLOUR_RGB('Opaque(160,160,160)', 0.09019608, 0.27058824, 0.51372549);
ENDSEC;
END-ISO-10303-21;
